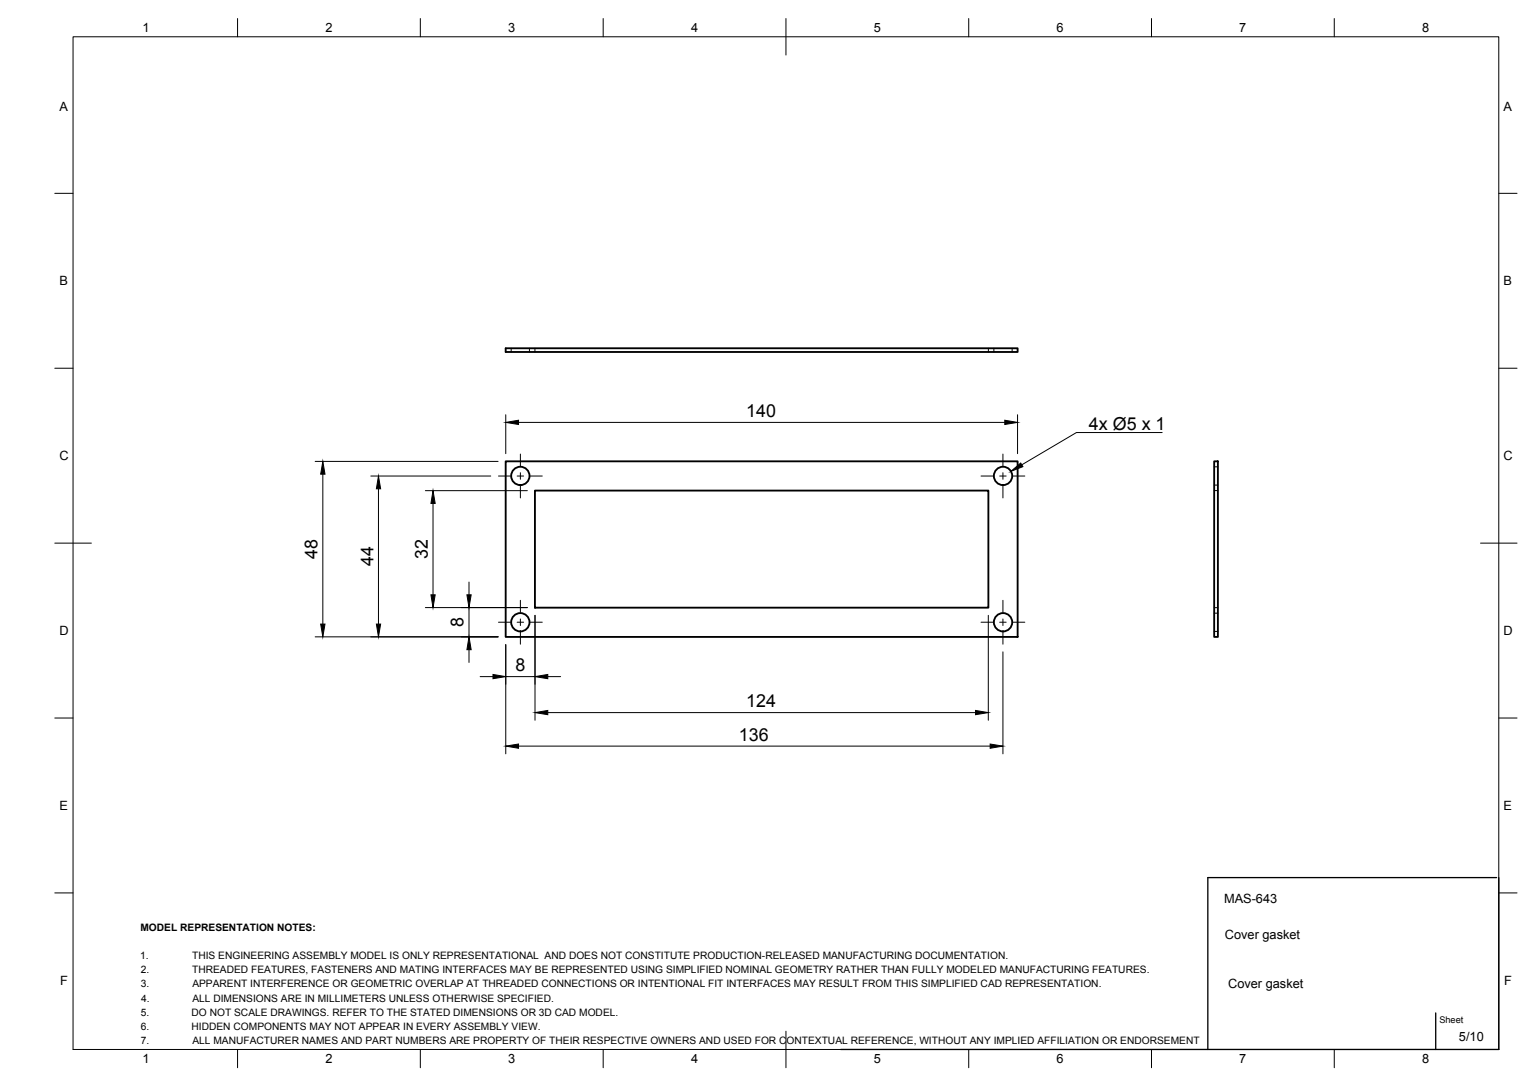
ISO-10303-21;
HEADER;
/* Generated by software containing ST-Developer
 * from STEP Tools, Inc. (www.steptools.com) 
 */

FILE_DESCRIPTION(
/* description */ ('Independent eighteen-tube parallel-flow evaporator geometry. Repeated
 machined headers and gasketed service covers, eighteen copper tubes, 
twenty-nine punched fins, threaded hose connections and bolted mountin
g feet. Native editable features and instanced parts. Braze details, w
orking fluid, pressure and thermal ratings require engineering selecti
on.'),
/* implementation_level */ '2;1');

FILE_NAME(
/* name */ 'Cover gasket.step',
/* time_stamp */ '2026-11-08T20:53:59-08:00',
/* author */ (''),
/* organization */ (''),
/* preprocessor_version */ 'ST-DEVELOPER v20.2',
/* originating_system */ 'Autodesk Translation Framework v15.17.0.0',
/* authorisation */ '');

FILE_SCHEMA (('AUTOMOTIVE_DESIGN { 1 0 10303 214 3 1 1 }'));
ENDSEC;

DATA;
#10=MECHANICAL_DESIGN_GEOMETRIC_PRESENTATION_REPRESENTATION('',(#335),#42620);
#315=SHAPE_REPRESENTATION_RELATIONSHIP('SRR','None',#42725,#325);
#325=ADVANCED_BREP_SHAPE_REPRESENTATION('',(#345),#42612);
#335=STYLED_ITEM('',(#42784),#345);
#345=MANIFOLD_SOLID_BREP('Body1',#10385);
#409=FACE_BOUND('',#1573,.T.);
#410=FACE_BOUND('',#1574,.T.);
#411=FACE_BOUND('',#1575,.T.);
#412=FACE_BOUND('',#1576,.T.);
#413=FACE_BOUND('',#1577,.T.);
#414=FACE_BOUND('',#1579,.T.);
#415=FACE_BOUND('',#1580,.T.);
#416=FACE_BOUND('',#1581,.T.);
#417=FACE_BOUND('',#1582,.T.);
#418=FACE_BOUND('',#1583,.T.);
#523=PLANE('',#10953);
#524=PLANE('',#10954);
#525=PLANE('',#10955);
#526=PLANE('',#10956);
#527=PLANE('',#10957);
#528=PLANE('',#10958);
#529=PLANE('',#10959);
#530=PLANE('',#10960);
#531=PLANE('',#10961);
#532=PLANE('',#10962);
#960=FACE_OUTER_BOUND('',#1560,.T.);
#961=FACE_OUTER_BOUND('',#1561,.T.);
#962=FACE_OUTER_BOUND('',#1562,.T.);
#963=FACE_OUTER_BOUND('',#1563,.T.);
#964=FACE_OUTER_BOUND('',#1564,.T.);
#965=FACE_OUTER_BOUND('',#1565,.T.);
#966=FACE_OUTER_BOUND('',#1566,.T.);
#967=FACE_OUTER_BOUND('',#1567,.T.);
#968=FACE_OUTER_BOUND('',#1568,.T.);
#969=FACE_OUTER_BOUND('',#1569,.T.);
#970=FACE_OUTER_BOUND('',#1570,.T.);
#971=FACE_OUTER_BOUND('',#1571,.T.);
#972=FACE_OUTER_BOUND('',#1572,.T.);
#973=FACE_OUTER_BOUND('',#1578,.T.);
#1560=EDGE_LOOP('',(#8459,#8460,#8461,#8462));
#1561=EDGE_LOOP('',(#8463,#8464,#8465,#8466));
#1562=EDGE_LOOP('',(#8467,#8468,#8469,#8470));
#1563=EDGE_LOOP('',(#8471,#8472,#8473,#8474));
#1564=EDGE_LOOP('',(#8475,#8476,#8477,#8478));
#1565=EDGE_LOOP('',(#8479,#8480,#8481,#8482));
#1566=EDGE_LOOP('',(#8483,#8484,#8485,#8486));
#1567=EDGE_LOOP('',(#8487,#8488,#8489,#8490));
#1568=EDGE_LOOP('',(#8491,#8492,#8493,#8494));
#1569=EDGE_LOOP('',(#8495,#8496,#8497,#8498));
#1570=EDGE_LOOP('',(#8499,#8500,#8501,#8502));
#1571=EDGE_LOOP('',(#8503,#8504,#8505,#8506));
#1572=EDGE_LOOP('',(#8507,#8508,#8509,#8510));
#1573=EDGE_LOOP('',(#8511,#8512,#8513,#8514));
#1574=EDGE_LOOP('',(#8515));
#1575=EDGE_LOOP('',(#8516));
#1576=EDGE_LOOP('',(#8517));
#1577=EDGE_LOOP('',(#8518));
#1578=EDGE_LOOP('',(#8519,#8520,#8521,#8522));
#1579=EDGE_LOOP('',(#8523,#8524,#8525,#8526));
#1580=EDGE_LOOP('',(#8527));
#1581=EDGE_LOOP('',(#8528));
#1582=EDGE_LOOP('',(#8529));
#1583=EDGE_LOOP('',(#8530));
#1919=CIRCLE('',#10942,2.5);
#1920=CIRCLE('',#10943,2.5);
#1921=CIRCLE('',#10945,2.5);
#1922=CIRCLE('',#10946,2.5);
#1923=CIRCLE('',#10948,2.5);
#1924=CIRCLE('',#10949,2.5);
#1925=CIRCLE('',#10951,2.5);
#1926=CIRCLE('',#10952,2.5);
#3134=LINE('',#34894,#3672);
#3135=LINE('',#34900,#3673);
#3136=LINE('',#34906,#3674);
#3137=LINE('',#34912,#3675);
#3138=LINE('',#34917,#3676);
#3139=LINE('',#34919,#3677);
#3140=LINE('',#34921,#3678);
#3141=LINE('',#34922,#3679);
#3142=LINE('',#34925,#3680);
#3143=LINE('',#34927,#3681);
#3144=LINE('',#34928,#3682);
#3145=LINE('',#34931,#3683);
#3146=LINE('',#34933,#3684);
#3147=LINE('',#34934,#3685);
#3148=LINE('',#34936,#3686);
#3149=LINE('',#34937,#3687);
#3150=LINE('',#34941,#3688);
#3151=LINE('',#34943,#3689);
#3152=LINE('',#34945,#3690);
#3153=LINE('',#34946,#3691);
#3154=LINE('',#34949,#3692);
#3155=LINE('',#34951,#3693);
#3156=LINE('',#34952,#3694);
#3157=LINE('',#34955,#3695);
#3158=LINE('',#34957,#3696);
#3159=LINE('',#34958,#3697);
#3160=LINE('',#34960,#3698);
#3161=LINE('',#34961,#3699);
#3672=VECTOR('',#12519,2.5);
#3673=VECTOR('',#12526,2.5);
#3674=VECTOR('',#12533,2.5);
#3675=VECTOR('',#12540,2.5);
#3676=VECTOR('',#12545,10.);
#3677=VECTOR('',#12546,10.);
#3678=VECTOR('',#12547,10.);
#3679=VECTOR('',#12548,10.);
#3680=VECTOR('',#12551,10.);
#3681=VECTOR('',#12552,10.);
#3682=VECTOR('',#12553,10.);
#3683=VECTOR('',#12556,10.);
#3684=VECTOR('',#12557,10.);
#3685=VECTOR('',#12558,10.);
#3686=VECTOR('',#12561,10.);
#3687=VECTOR('',#12562,10.);
#3688=VECTOR('',#12565,10.);
#3689=VECTOR('',#12566,10.);
#3690=VECTOR('',#12567,10.);
#3691=VECTOR('',#12568,10.);
#3692=VECTOR('',#12571,10.);
#3693=VECTOR('',#12572,10.);
#3694=VECTOR('',#12573,10.);
#3695=VECTOR('',#12576,10.);
#3696=VECTOR('',#12577,10.);
#3697=VECTOR('',#12578,10.);
#3698=VECTOR('',#12581,10.);
#3699=VECTOR('',#12582,10.);
#4559=VERTEX_POINT('',#34891);
#4560=VERTEX_POINT('',#34893);
#4561=VERTEX_POINT('',#34897);
#4562=VERTEX_POINT('',#34899);
#4563=VERTEX_POINT('',#34903);
#4564=VERTEX_POINT('',#34905);
#4565=VERTEX_POINT('',#34909);
#4566=VERTEX_POINT('',#34911);
#4567=VERTEX_POINT('',#34915);
#4568=VERTEX_POINT('',#34916);
#4569=VERTEX_POINT('',#34918);
#4570=VERTEX_POINT('',#34920);
#4571=VERTEX_POINT('',#34924);
#4572=VERTEX_POINT('',#34926);
#4573=VERTEX_POINT('',#34930);
#4574=VERTEX_POINT('',#34932);
#4575=VERTEX_POINT('',#34939);
#4576=VERTEX_POINT('',#34940);
#4577=VERTEX_POINT('',#34942);
#4578=VERTEX_POINT('',#34944);
#4579=VERTEX_POINT('',#34948);
#4580=VERTEX_POINT('',#34950);
#4581=VERTEX_POINT('',#34954);
#4582=VERTEX_POINT('',#34956);
#5912=EDGE_CURVE('',#4559,#4559,#1919,.T.);
#5913=EDGE_CURVE('',#4559,#4560,#3134,.T.);
#5914=EDGE_CURVE('',#4560,#4560,#1920,.T.);
#5915=EDGE_CURVE('',#4561,#4561,#1921,.T.);
#5916=EDGE_CURVE('',#4561,#4562,#3135,.T.);
#5917=EDGE_CURVE('',#4562,#4562,#1922,.T.);
#5918=EDGE_CURVE('',#4563,#4563,#1923,.T.);
#5919=EDGE_CURVE('',#4563,#4564,#3136,.T.);
#5920=EDGE_CURVE('',#4564,#4564,#1924,.T.);
#5921=EDGE_CURVE('',#4565,#4565,#1925,.T.);
#5922=EDGE_CURVE('',#4565,#4566,#3137,.T.);
#5923=EDGE_CURVE('',#4566,#4566,#1926,.T.);
#5924=EDGE_CURVE('',#4567,#4568,#3138,.T.);
#5925=EDGE_CURVE('',#4567,#4569,#3139,.T.);
#5926=EDGE_CURVE('',#4570,#4569,#3140,.T.);
#5927=EDGE_CURVE('',#4568,#4570,#3141,.T.);
#5928=EDGE_CURVE('',#4571,#4567,#3142,.T.);
#5929=EDGE_CURVE('',#4571,#4572,#3143,.T.);
#5930=EDGE_CURVE('',#4569,#4572,#3144,.T.);
#5931=EDGE_CURVE('',#4573,#4571,#3145,.T.);
#5932=EDGE_CURVE('',#4573,#4574,#3146,.T.);
#5933=EDGE_CURVE('',#4572,#4574,#3147,.T.);
#5934=EDGE_CURVE('',#4568,#4573,#3148,.T.);
#5935=EDGE_CURVE('',#4574,#4570,#3149,.T.);
#5936=EDGE_CURVE('',#4575,#4576,#3150,.T.);
#5937=EDGE_CURVE('',#4576,#4577,#3151,.T.);
#5938=EDGE_CURVE('',#4578,#4577,#3152,.T.);
#5939=EDGE_CURVE('',#4575,#4578,#3153,.T.);
#5940=EDGE_CURVE('',#4579,#4575,#3154,.T.);
#5941=EDGE_CURVE('',#4580,#4578,#3155,.T.);
#5942=EDGE_CURVE('',#4579,#4580,#3156,.T.);
#5943=EDGE_CURVE('',#4581,#4579,#3157,.T.);
#5944=EDGE_CURVE('',#4582,#4580,#3158,.T.);
#5945=EDGE_CURVE('',#4581,#4582,#3159,.T.);
#5946=EDGE_CURVE('',#4576,#4581,#3160,.T.);
#5947=EDGE_CURVE('',#4577,#4582,#3161,.T.);
#8459=ORIENTED_EDGE('',*,*,#5912,.F.);
#8460=ORIENTED_EDGE('',*,*,#5913,.T.);
#8461=ORIENTED_EDGE('',*,*,#5914,.F.);
#8462=ORIENTED_EDGE('',*,*,#5913,.F.);
#8463=ORIENTED_EDGE('',*,*,#5915,.F.);
#8464=ORIENTED_EDGE('',*,*,#5916,.T.);
#8465=ORIENTED_EDGE('',*,*,#5917,.F.);
#8466=ORIENTED_EDGE('',*,*,#5916,.F.);
#8467=ORIENTED_EDGE('',*,*,#5918,.F.);
#8468=ORIENTED_EDGE('',*,*,#5919,.T.);
#8469=ORIENTED_EDGE('',*,*,#5920,.F.);
#8470=ORIENTED_EDGE('',*,*,#5919,.F.);
#8471=ORIENTED_EDGE('',*,*,#5921,.F.);
#8472=ORIENTED_EDGE('',*,*,#5922,.T.);
#8473=ORIENTED_EDGE('',*,*,#5923,.F.);
#8474=ORIENTED_EDGE('',*,*,#5922,.F.);
#8475=ORIENTED_EDGE('',*,*,#5924,.F.);
#8476=ORIENTED_EDGE('',*,*,#5925,.T.);
#8477=ORIENTED_EDGE('',*,*,#5926,.F.);
#8478=ORIENTED_EDGE('',*,*,#5927,.F.);
#8479=ORIENTED_EDGE('',*,*,#5928,.F.);
#8480=ORIENTED_EDGE('',*,*,#5929,.T.);
#8481=ORIENTED_EDGE('',*,*,#5930,.F.);
#8482=ORIENTED_EDGE('',*,*,#5925,.F.);
#8483=ORIENTED_EDGE('',*,*,#5931,.F.);
#8484=ORIENTED_EDGE('',*,*,#5932,.T.);
#8485=ORIENTED_EDGE('',*,*,#5933,.F.);
#8486=ORIENTED_EDGE('',*,*,#5929,.F.);
#8487=ORIENTED_EDGE('',*,*,#5934,.F.);
#8488=ORIENTED_EDGE('',*,*,#5927,.T.);
#8489=ORIENTED_EDGE('',*,*,#5935,.F.);
#8490=ORIENTED_EDGE('',*,*,#5932,.F.);
#8491=ORIENTED_EDGE('',*,*,#5936,.T.);
#8492=ORIENTED_EDGE('',*,*,#5937,.T.);
#8493=ORIENTED_EDGE('',*,*,#5938,.F.);
#8494=ORIENTED_EDGE('',*,*,#5939,.F.);
#8495=ORIENTED_EDGE('',*,*,#5940,.T.);
#8496=ORIENTED_EDGE('',*,*,#5939,.T.);
#8497=ORIENTED_EDGE('',*,*,#5941,.F.);
#8498=ORIENTED_EDGE('',*,*,#5942,.F.);
#8499=ORIENTED_EDGE('',*,*,#5943,.T.);
#8500=ORIENTED_EDGE('',*,*,#5942,.T.);
#8501=ORIENTED_EDGE('',*,*,#5944,.F.);
#8502=ORIENTED_EDGE('',*,*,#5945,.F.);
#8503=ORIENTED_EDGE('',*,*,#5946,.T.);
#8504=ORIENTED_EDGE('',*,*,#5945,.T.);
#8505=ORIENTED_EDGE('',*,*,#5947,.F.);
#8506=ORIENTED_EDGE('',*,*,#5937,.F.);
#8507=ORIENTED_EDGE('',*,*,#5947,.T.);
#8508=ORIENTED_EDGE('',*,*,#5944,.T.);
#8509=ORIENTED_EDGE('',*,*,#5941,.T.);
#8510=ORIENTED_EDGE('',*,*,#5938,.T.);
#8511=ORIENTED_EDGE('',*,*,#5924,.T.);
#8512=ORIENTED_EDGE('',*,*,#5934,.T.);
#8513=ORIENTED_EDGE('',*,*,#5931,.T.);
#8514=ORIENTED_EDGE('',*,*,#5928,.T.);
#8515=ORIENTED_EDGE('',*,*,#5921,.T.);
#8516=ORIENTED_EDGE('',*,*,#5918,.T.);
#8517=ORIENTED_EDGE('',*,*,#5915,.T.);
#8518=ORIENTED_EDGE('',*,*,#5912,.T.);
#8519=ORIENTED_EDGE('',*,*,#5946,.F.);
#8520=ORIENTED_EDGE('',*,*,#5936,.F.);
#8521=ORIENTED_EDGE('',*,*,#5940,.F.);
#8522=ORIENTED_EDGE('',*,*,#5943,.F.);
#8523=ORIENTED_EDGE('',*,*,#5926,.T.);
#8524=ORIENTED_EDGE('',*,*,#5930,.T.);
#8525=ORIENTED_EDGE('',*,*,#5933,.T.);
#8526=ORIENTED_EDGE('',*,*,#5935,.T.);
#8527=ORIENTED_EDGE('',*,*,#5923,.T.);
#8528=ORIENTED_EDGE('',*,*,#5920,.T.);
#8529=ORIENTED_EDGE('',*,*,#5917,.T.);
#8530=ORIENTED_EDGE('',*,*,#5914,.T.);
#9716=CYLINDRICAL_SURFACE('',#10941,2.5);
#9717=CYLINDRICAL_SURFACE('',#10944,2.5);
#9718=CYLINDRICAL_SURFACE('',#10947,2.5);
#9719=CYLINDRICAL_SURFACE('',#10950,2.5);
#10196=ADVANCED_FACE('',(#960),#9716,.F.);
#10197=ADVANCED_FACE('',(#961),#9717,.F.);
#10198=ADVANCED_FACE('',(#962),#9718,.F.);
#10199=ADVANCED_FACE('',(#963),#9719,.F.);
#10200=ADVANCED_FACE('',(#964),#523,.F.);
#10201=ADVANCED_FACE('',(#965),#524,.F.);
#10202=ADVANCED_FACE('',(#966),#525,.F.);
#10203=ADVANCED_FACE('',(#967),#526,.F.);
#10204=ADVANCED_FACE('',(#968),#527,.T.);
#10205=ADVANCED_FACE('',(#969),#528,.T.);
#10206=ADVANCED_FACE('',(#970),#529,.T.);
#10207=ADVANCED_FACE('',(#971),#530,.T.);
#10208=ADVANCED_FACE('',(#972,#409,#410,#411,#412,#413),#531,.T.);
#10209=ADVANCED_FACE('',(#973,#414,#415,#416,#417,#418),#532,.F.);
#10385=CLOSED_SHELL('',(#10196,#10197,#10198,#10199,#10200,#10201,#10202,
#10203,#10204,#10205,#10206,#10207,#10208,#10209));
#10940=AXIS2_PLACEMENT_3D('',#34889,#12513,#12514);
#10941=AXIS2_PLACEMENT_3D('',#34890,#12515,#12516);
#10942=AXIS2_PLACEMENT_3D('',#34892,#12517,#12518);
#10943=AXIS2_PLACEMENT_3D('',#34895,#12520,#12521);
#10944=AXIS2_PLACEMENT_3D('',#34896,#12522,#12523);
#10945=AXIS2_PLACEMENT_3D('',#34898,#12524,#12525);
#10946=AXIS2_PLACEMENT_3D('',#34901,#12527,#12528);
#10947=AXIS2_PLACEMENT_3D('',#34902,#12529,#12530);
#10948=AXIS2_PLACEMENT_3D('',#34904,#12531,#12532);
#10949=AXIS2_PLACEMENT_3D('',#34907,#12534,#12535);
#10950=AXIS2_PLACEMENT_3D('',#34908,#12536,#12537);
#10951=AXIS2_PLACEMENT_3D('',#34910,#12538,#12539);
#10952=AXIS2_PLACEMENT_3D('',#34913,#12541,#12542);
#10953=AXIS2_PLACEMENT_3D('',#34914,#12543,#12544);
#10954=AXIS2_PLACEMENT_3D('',#34923,#12549,#12550);
#10955=AXIS2_PLACEMENT_3D('',#34929,#12554,#12555);
#10956=AXIS2_PLACEMENT_3D('',#34935,#12559,#12560);
#10957=AXIS2_PLACEMENT_3D('',#34938,#12563,#12564);
#10958=AXIS2_PLACEMENT_3D('',#34947,#12569,#12570);
#10959=AXIS2_PLACEMENT_3D('',#34953,#12574,#12575);
#10960=AXIS2_PLACEMENT_3D('',#34959,#12579,#12580);
#10961=AXIS2_PLACEMENT_3D('',#34962,#12583,#12584);
#10962=AXIS2_PLACEMENT_3D('',#34963,#12585,#12586);
#12513=DIRECTION('axis',(0.,0.,1.));
#12514=DIRECTION('refdir',(1.,0.,0.));
#12515=DIRECTION('center_axis',(0.,0.,-1.));
#12516=DIRECTION('ref_axis',(1.,0.,0.));
#12517=DIRECTION('center_axis',(0.,0.,-1.));
#12518=DIRECTION('ref_axis',(1.,0.,0.));
#12519=DIRECTION('',(0.,0.,-1.));
#12520=DIRECTION('center_axis',(0.,0.,1.));
#12521=DIRECTION('ref_axis',(1.,0.,0.));
#12522=DIRECTION('center_axis',(0.,0.,-1.));
#12523=DIRECTION('ref_axis',(1.,0.,0.));
#12524=DIRECTION('center_axis',(0.,0.,-1.));
#12525=DIRECTION('ref_axis',(1.,0.,0.));
#12526=DIRECTION('',(0.,0.,-1.));
#12527=DIRECTION('center_axis',(0.,0.,1.));
#12528=DIRECTION('ref_axis',(1.,0.,0.));
#12529=DIRECTION('center_axis',(0.,0.,-1.));
#12530=DIRECTION('ref_axis',(1.,0.,0.));
#12531=DIRECTION('center_axis',(0.,0.,-1.));
#12532=DIRECTION('ref_axis',(1.,0.,0.));
#12533=DIRECTION('',(0.,0.,-1.));
#12534=DIRECTION('center_axis',(0.,0.,1.));
#12535=DIRECTION('ref_axis',(1.,0.,0.));
#12536=DIRECTION('center_axis',(0.,0.,-1.));
#12537=DIRECTION('ref_axis',(1.,0.,0.));
#12538=DIRECTION('center_axis',(0.,0.,-1.));
#12539=DIRECTION('ref_axis',(1.,0.,0.));
#12540=DIRECTION('',(0.,0.,-1.));
#12541=DIRECTION('center_axis',(0.,0.,1.));
#12542=DIRECTION('ref_axis',(1.,0.,0.));
#12543=DIRECTION('center_axis',(0.,-1.,0.));
#12544=DIRECTION('ref_axis',(-1.,0.,0.));
#12545=DIRECTION('',(-1.,0.,0.));
#12546=DIRECTION('',(0.,0.,-1.));
#12547=DIRECTION('',(1.,0.,0.));
#12548=DIRECTION('',(0.,0.,-1.));
#12549=DIRECTION('center_axis',(1.,0.,0.));
#12550=DIRECTION('ref_axis',(0.,-1.,0.));
#12551=DIRECTION('',(0.,-1.,0.));
#12552=DIRECTION('',(0.,0.,-1.));
#12553=DIRECTION('',(0.,1.,0.));
#12554=DIRECTION('center_axis',(0.,1.,0.));
#12555=DIRECTION('ref_axis',(1.,0.,0.));
#12556=DIRECTION('',(1.,0.,0.));
#12557=DIRECTION('',(0.,0.,-1.));
#12558=DIRECTION('',(-1.,0.,0.));
#12559=DIRECTION('center_axis',(-1.,0.,0.));
#12560=DIRECTION('ref_axis',(0.,1.,0.));
#12561=DIRECTION('',(0.,1.,0.));
#12562=DIRECTION('',(0.,-1.,0.));
#12563=DIRECTION('center_axis',(0.,1.,0.));
#12564=DIRECTION('ref_axis',(-1.,0.,0.));
#12565=DIRECTION('',(-1.,0.,0.));
#12566=DIRECTION('',(0.,0.,1.));
#12567=DIRECTION('',(-1.,0.,0.));
#12568=DIRECTION('',(0.,0.,1.));
#12569=DIRECTION('center_axis',(1.,0.,0.));
#12570=DIRECTION('ref_axis',(0.,1.,0.));
#12571=DIRECTION('',(0.,1.,0.));
#12572=DIRECTION('',(0.,1.,0.));
#12573=DIRECTION('',(0.,0.,1.));
#12574=DIRECTION('center_axis',(0.,-1.,0.));
#12575=DIRECTION('ref_axis',(1.,0.,0.));
#12576=DIRECTION('',(1.,0.,0.));
#12577=DIRECTION('',(1.,0.,0.));
#12578=DIRECTION('',(0.,0.,1.));
#12579=DIRECTION('center_axis',(-1.,0.,0.));
#12580=DIRECTION('ref_axis',(0.,-1.,0.));
#12581=DIRECTION('',(0.,-1.,0.));
#12582=DIRECTION('',(0.,-1.,0.));
#12583=DIRECTION('center_axis',(0.,0.,1.));
#12584=DIRECTION('ref_axis',(1.,0.,0.));
#12585=DIRECTION('center_axis',(0.,0.,1.));
#12586=DIRECTION('ref_axis',(1.,0.,0.));
#34889=CARTESIAN_POINT('',(0.,0.,0.));
#34890=CARTESIAN_POINT('Origin',(20.,-66.,36.5));
#34891=CARTESIAN_POINT('',(17.5,-66.,37.));
#34892=CARTESIAN_POINT('Origin',(20.,-66.,37.));
#34893=CARTESIAN_POINT('',(17.5,-66.,36.));
#34894=CARTESIAN_POINT('',(17.5,-66.,36.5));
#34895=CARTESIAN_POINT('Origin',(20.,-66.,36.));
#34896=CARTESIAN_POINT('Origin',(-20.,-66.,36.5));
#34897=CARTESIAN_POINT('',(-22.5,-66.,37.));
#34898=CARTESIAN_POINT('Origin',(-20.,-66.,37.));
#34899=CARTESIAN_POINT('',(-22.5,-66.,36.));
#34900=CARTESIAN_POINT('',(-22.5,-66.,36.5));
#34901=CARTESIAN_POINT('Origin',(-20.,-66.,36.));
#34902=CARTESIAN_POINT('Origin',(-20.,66.,36.5));
#34903=CARTESIAN_POINT('',(-22.5,66.,37.));
#34904=CARTESIAN_POINT('Origin',(-20.,66.,37.));
#34905=CARTESIAN_POINT('',(-22.5,66.,36.));
#34906=CARTESIAN_POINT('',(-22.5,66.,36.5));
#34907=CARTESIAN_POINT('Origin',(-20.,66.,36.));
#34908=CARTESIAN_POINT('Origin',(20.,66.,36.5));
#34909=CARTESIAN_POINT('',(17.5,66.,37.));
#34910=CARTESIAN_POINT('Origin',(20.,66.,37.));
#34911=CARTESIAN_POINT('',(17.5,66.,36.));
#34912=CARTESIAN_POINT('',(17.5,66.,36.5));
#34913=CARTESIAN_POINT('Origin',(20.,66.,36.));
#34914=CARTESIAN_POINT('Origin',(16.,-62.,37.));
#34915=CARTESIAN_POINT('',(16.,-62.,37.));
#34916=CARTESIAN_POINT('',(-16.,-62.,37.));
#34917=CARTESIAN_POINT('',(8.,-62.,37.));
#34918=CARTESIAN_POINT('',(16.,-62.,36.));
#34919=CARTESIAN_POINT('',(16.,-62.,37.));
#34920=CARTESIAN_POINT('',(-16.,-62.,36.));
#34921=CARTESIAN_POINT('',(8.,-62.,36.));
#34922=CARTESIAN_POINT('',(-16.,-62.,37.));
#34923=CARTESIAN_POINT('Origin',(16.,62.,37.));
#34924=CARTESIAN_POINT('',(16.,62.,37.));
#34925=CARTESIAN_POINT('',(16.,31.,37.));
#34926=CARTESIAN_POINT('',(16.,62.,36.));
#34927=CARTESIAN_POINT('',(16.,62.,37.));
#34928=CARTESIAN_POINT('',(16.,31.,36.));
#34929=CARTESIAN_POINT('Origin',(-16.,62.,37.));
#34930=CARTESIAN_POINT('',(-16.,62.,37.));
#34931=CARTESIAN_POINT('',(-8.,62.,37.));
#34932=CARTESIAN_POINT('',(-16.,62.,36.));
#34933=CARTESIAN_POINT('',(-16.,62.,37.));
#34934=CARTESIAN_POINT('',(-8.,62.,36.));
#34935=CARTESIAN_POINT('Origin',(-16.,-62.,37.));
#34936=CARTESIAN_POINT('',(-16.,-31.,37.));
#34937=CARTESIAN_POINT('',(-16.,-31.,36.));
#34938=CARTESIAN_POINT('Origin',(24.,70.,36.));
#34939=CARTESIAN_POINT('',(24.,70.,36.));
#34940=CARTESIAN_POINT('',(-24.,70.,36.));
#34941=CARTESIAN_POINT('',(24.,70.,36.));
#34942=CARTESIAN_POINT('',(-24.,70.,37.));
#34943=CARTESIAN_POINT('',(-24.,70.,36.));
#34944=CARTESIAN_POINT('',(24.,70.,37.));
#34945=CARTESIAN_POINT('',(24.,70.,37.));
#34946=CARTESIAN_POINT('',(24.,70.,36.));
#34947=CARTESIAN_POINT('Origin',(24.,-70.,36.));
#34948=CARTESIAN_POINT('',(24.,-70.,36.));
#34949=CARTESIAN_POINT('',(24.,-70.,36.));
#34950=CARTESIAN_POINT('',(24.,-70.,37.));
#34951=CARTESIAN_POINT('',(24.,-70.,37.));
#34952=CARTESIAN_POINT('',(24.,-70.,36.));
#34953=CARTESIAN_POINT('Origin',(-24.,-70.,36.));
#34954=CARTESIAN_POINT('',(-24.,-70.,36.));
#34955=CARTESIAN_POINT('',(-24.,-70.,36.));
#34956=CARTESIAN_POINT('',(-24.,-70.,37.));
#34957=CARTESIAN_POINT('',(-24.,-70.,37.));
#34958=CARTESIAN_POINT('',(-24.,-70.,36.));
#34959=CARTESIAN_POINT('Origin',(-24.,70.,36.));
#34960=CARTESIAN_POINT('',(-24.,70.,36.));
#34961=CARTESIAN_POINT('',(-24.,70.,37.));
#34962=CARTESIAN_POINT('Origin',(0.,0.,37.));
#34963=CARTESIAN_POINT('Origin',(0.,0.,36.));
#42600=UNCERTAINTY_MEASURE_WITH_UNIT(LENGTH_MEASURE(0.01),#42621,
'DISTANCE_ACCURACY_VALUE',
'Maximum model space distance between geometric entities at asserted c
onnectivities');
#42608=UNCERTAINTY_MEASURE_WITH_UNIT(LENGTH_MEASURE(0.01),#42621,
'DISTANCE_ACCURACY_VALUE',
'Maximum model space distance between geometric entities at asserted c
onnectivities');
#42612=(
GEOMETRIC_REPRESENTATION_CONTEXT(3)
GLOBAL_UNCERTAINTY_ASSIGNED_CONTEXT((#42600))
GLOBAL_UNIT_ASSIGNED_CONTEXT((#42621,#42623,#42624))
REPRESENTATION_CONTEXT('','3D')
);
#42620=(
GEOMETRIC_REPRESENTATION_CONTEXT(3)
GLOBAL_UNCERTAINTY_ASSIGNED_CONTEXT((#42608))
GLOBAL_UNIT_ASSIGNED_CONTEXT((#42621,#42623,#42624))
REPRESENTATION_CONTEXT('','3D')
);
#42621=(
LENGTH_UNIT()
NAMED_UNIT(*)
SI_UNIT(.MILLI.,.METRE.)
);
#42623=(
NAMED_UNIT(*)
PLANE_ANGLE_UNIT()
SI_UNIT($,.RADIAN.)
);
#42624=(
NAMED_UNIT(*)
SI_UNIT($,.STERADIAN.)
SOLID_ANGLE_UNIT()
);
#42628=SHAPE_DEFINITION_REPRESENTATION(#42639,#42725);
#42639=PRODUCT_DEFINITION_SHAPE('',$,#42737);
#42725=SHAPE_REPRESENTATION('',(#10940),#42612);
#42733=PRODUCT_DEFINITION_CONTEXT('part definition',#42768,'design');
#42737=PRODUCT_DEFINITION('Cover gasket','Cover gasket',#42748,#42733);
#42748=PRODUCT_DEFINITION_FORMATION('',$,#42773);
#42768=APPLICATION_CONTEXT(
'Core Data for Automotive Mechanical Design Process');
#42769=PRODUCT_CONTEXT('part definition',#42768,'mechanical');
#42773=PRODUCT('Cover gasket','Cover gasket',$,(#42769));
#42784=PRESENTATION_STYLE_ASSIGNMENT((#42792));
#42792=SURFACE_STYLE_USAGE(.BOTH.,#42800);
#42800=SURFACE_SIDE_STYLE('',(#42808));
#42808=SURFACE_STYLE_FILL_AREA(#42816);
#42816=FILL_AREA_STYLE('Dark gray',(#42824));
#42824=FILL_AREA_STYLE_COLOUR('Dark gray',#42832);
#42832=COLOUR_RGB('Dark gray',0.250980392156863,0.282352941176471,0.32156862745098);
ENDSEC;
END-ISO-10303-21;
